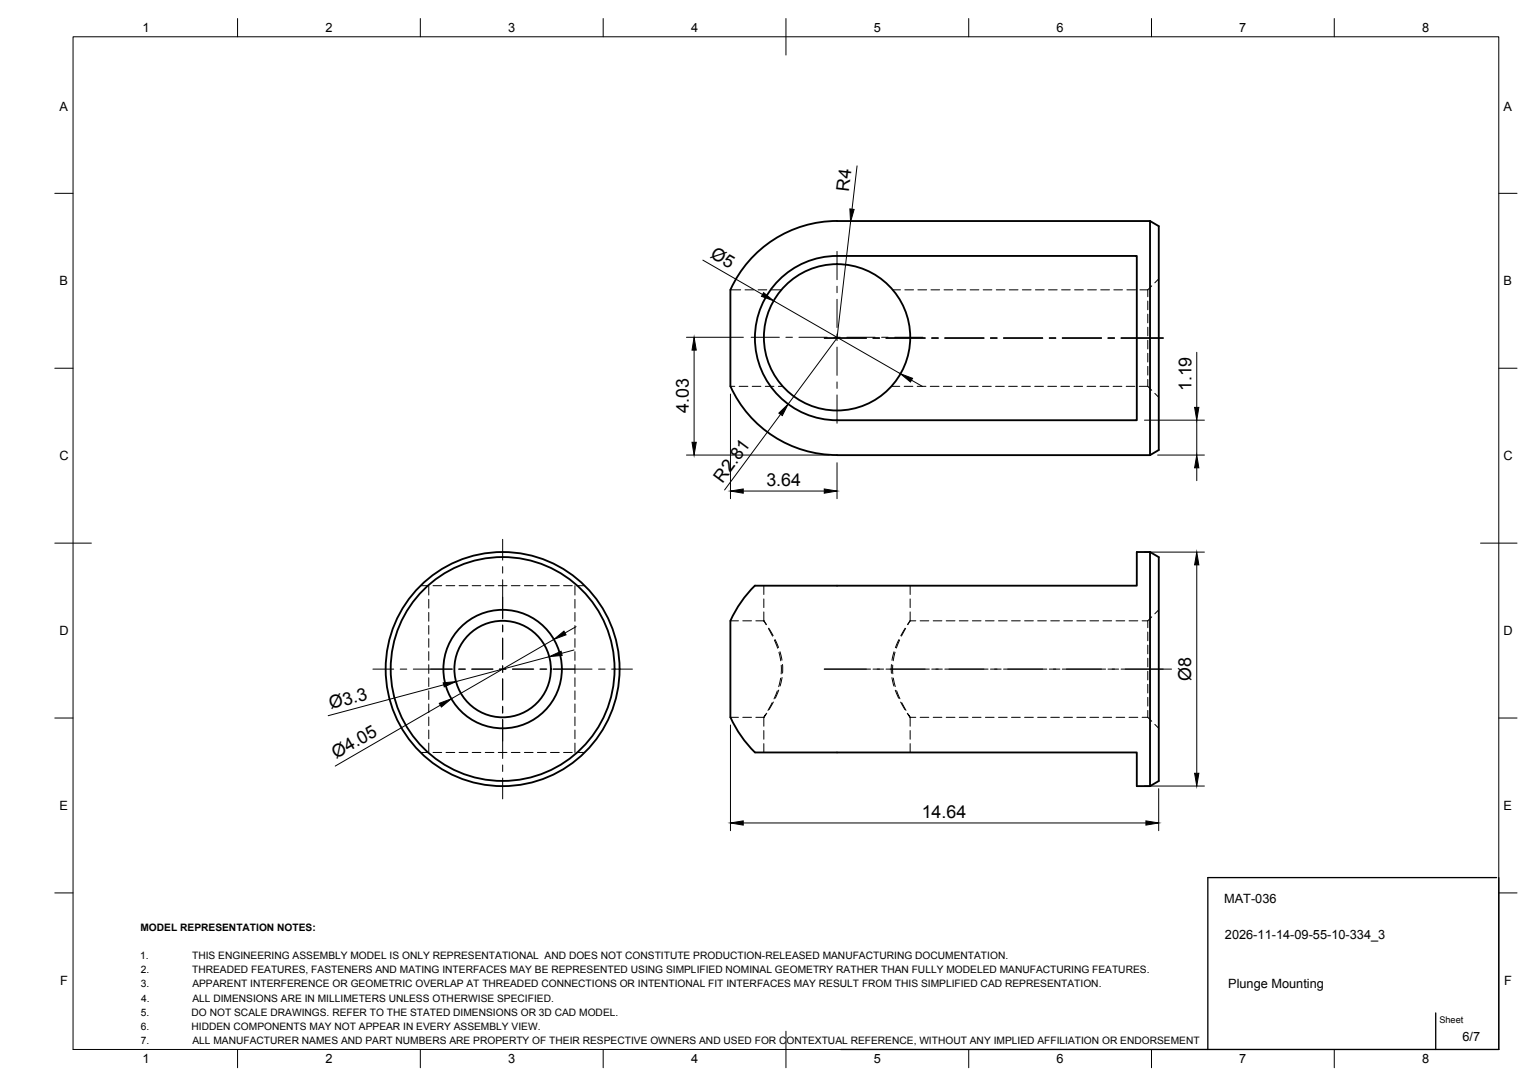
ISO-10303-21;
HEADER;
/* Generated by software containing ST-Developer
 * from STEP Tools, Inc. (www.steptools.com) 
 */

FILE_DESCRIPTION(
/* description */ (''),
/* implementation_level */ '2;1');

FILE_NAME(
/* name */ 'Plunge Mounting.step',
/* time_stamp */ '2026-11-14T09:55:16-08:00',
/* author */ (''),
/* organization */ (''),
/* preprocessor_version */ 'ST-DEVELOPER v20.2',
/* originating_system */ 'Autodesk Translation Framework v15.17.0.0',
/* authorisation */ '');

FILE_SCHEMA (('AUTOMOTIVE_DESIGN { 1 0 10303 214 3 1 1 }'));
ENDSEC;

DATA;
#10=MECHANICAL_DESIGN_GEOMETRIC_PRESENTATION_REPRESENTATION('',(#61),#170250);
#35=SPHERICAL_SURFACE('',#77715,4.00000000000002);
#47=SHAPE_REPRESENTATION_RELATIONSHIP('SRR','None',#170279,#53);
#53=ADVANCED_BREP_SHAPE_REPRESENTATION('',(#67),#170247);
#61=STYLED_ITEM('',(#170315),#67);
#67=MANIFOLD_SOLID_BREP('Body1',#71401);
#80=FACE_BOUND('',#15903,.T.);
#81=FACE_BOUND('',#15905,.T.);
#82=FACE_BOUND('',#15911,.T.);
#83=FACE_BOUND('',#15916,.T.);
#84=FACE_BOUND('',#15918,.T.);
#103=PLANE('',#77733);
#104=PLANE('',#77734);
#105=PLANE('',#77735);
#106=PLANE('',#77737);
#107=PLANE('',#77738);
#5376=CYLINDRICAL_SURFACE('',#77712,2.5);
#5377=CYLINDRICAL_SURFACE('',#77722,4.);
#5378=CYLINDRICAL_SURFACE('',#77732,1.65);
#5379=CYLINDRICAL_SURFACE('',#77736,1.65);
#10627=FACE_OUTER_BOUND('',#15902,.T.);
#10628=FACE_OUTER_BOUND('',#15904,.T.);
#10629=FACE_OUTER_BOUND('',#15906,.T.);
#10630=FACE_OUTER_BOUND('',#15907,.T.);
#10631=FACE_OUTER_BOUND('',#15908,.T.);
#10632=FACE_OUTER_BOUND('',#15909,.T.);
#10633=FACE_OUTER_BOUND('',#15910,.T.);
#10634=FACE_OUTER_BOUND('',#15912,.T.);
#10635=FACE_OUTER_BOUND('',#15913,.T.);
#10636=FACE_OUTER_BOUND('',#15914,.T.);
#10637=FACE_OUTER_BOUND('',#15915,.T.);
#10638=FACE_OUTER_BOUND('',#15917,.T.);
#15902=EDGE_LOOP('',(#65902,#65903,#65904,#65905,#65906,#65907,#65908,#65909,
#65910));
#15903=EDGE_LOOP('',(#65911,#65912));
#15904=EDGE_LOOP('',(#65913,#65914,#65915,#65916,#65917));
#15905=EDGE_LOOP('',(#65918));
#15906=EDGE_LOOP('',(#65919,#65920,#65921,#65922,#65923,#65924,#65925,#65926,
#65927,#65928,#65929,#65930,#65931));
#15907=EDGE_LOOP('',(#65932,#65933,#65934,#65935));
#15908=EDGE_LOOP('',(#65936,#65937,#65938,#65939,#65940));
#15909=EDGE_LOOP('',(#65941,#65942,#65943,#65944,#65945));
#15910=EDGE_LOOP('',(#65946));
#15911=EDGE_LOOP('',(#65947));
#15912=EDGE_LOOP('',(#65948,#65949));
#15913=EDGE_LOOP('',(#65950,#65951));
#15914=EDGE_LOOP('',(#65952,#65953,#65954,#65955,#65956,#65957));
#15915=EDGE_LOOP('',(#65958,#65959,#65960,#65961));
#15916=EDGE_LOOP('',(#65962));
#15917=EDGE_LOOP('',(#65963,#65964,#65965,#65966));
#15918=EDGE_LOOP('',(#65967));
#21024=CIRCLE('',#77713,2.5);
#21025=CIRCLE('',#77714,2.5);
#21026=CIRCLE('',#77716,3.9999999997442);
#21027=CIRCLE('',#77717,2.80668844013728);
#21028=CIRCLE('',#77718,3.9999999997442);
#21029=CIRCLE('',#77719,3.9999999997442);
#21030=CIRCLE('',#77720,2.80668844013726);
#21031=CIRCLE('',#77721,1.64999996202742);
#21032=CIRCLE('',#77723,4.);
#21033=CIRCLE('',#77724,4.);
#21034=CIRCLE('',#77725,4.);
#21035=CIRCLE('',#77726,4.);
#21036=CIRCLE('',#77728,1.65);
#21037=CIRCLE('',#77729,2.025);
#21038=CIRCLE('',#77731,3.826794919);
#24347=B_SPLINE_CURVE_WITH_KNOTS('',3,(#169973,#169974,#169975,#169976,
#169977,#169978,#169979,#169980,#169981,#169982,#169983,#169984,#169985,
#169986,#169987,#169988,#169989,#169990),.UNSPECIFIED.,.F.,.F.,(4,2,2,2,
2,2,2,2,4),(-0.772891272014126,-0.711371011943309,-0.647238677062543,-0.582315553959231,
-0.517392430855918,-0.452469307752605,-0.387546184649291,-0.323413849768526,
-0.261893589697701),.UNSPECIFIED.);
#24348=B_SPLINE_CURVE_WITH_KNOTS('',3,(#169995,#169996,#169997,#169998),
 .UNSPECIFIED.,.F.,.F.,(4,4),(-0.261893589697701,-0.25928151488776),
 .UNSPECIFIED.);
#24349=B_SPLINE_CURVE_WITH_KNOTS('',3,(#169999,#170000,#170001,#170002,
#170003,#170004,#170005,#170006,#170007,#170008,#170009,#170010,#170011,
#170012,#170013,#170014,#170015,#170016,#170017,#170018,#170019),
 .UNSPECIFIED.,.F.,.F.,(4,2,2,2,3,2,2,2,2,4),(-0.25928151488776,-0.194741358681164,
-0.130201202474569,-0.0651006012372844,0.,0.0651006012372838,0.130201202474568,
0.194741358681163,0.259281514887759,0.261893589697708),.UNSPECIFIED.);
#24350=B_SPLINE_CURVE_WITH_KNOTS('',3,(#170022,#170023,#170024,#170025,
#170026,#170027,#170028,#170029,#170030,#170031),.UNSPECIFIED.,.F.,.F.,
(4,2,2,2,4),(-0.772891272014128,-0.711371011943309,-0.647238677062543,-0.58231555395923,
-0.517392430855917),.UNSPECIFIED.);
#24351=B_SPLINE_CURVE_WITH_KNOTS('',3,(#170032,#170033,#170034,#170035,
#170036,#170037,#170038,#170039,#170040,#170041,#170042,#170043,#170044,
#170045,#170046,#170047,#170048,#170049,#170050,#170051,#170052,#170053,
#170054,#170055,#170056,#170057,#170058,#170059,#170060),.UNSPECIFIED.,
 .F.,.F.,(4,2,2,2,2,2,2,2,3,2,2,2,2,4),(-0.517392430855917,-0.452469307752604,
-0.38754618464929,-0.323413849768524,-0.259281514887758,-0.194741358681163,
-0.130201202474568,-0.0651006012372838,0.,0.0651694580098041,0.130338916019608,
0.194810907043524,0.25928289806744,0.261894972877388),.UNSPECIFIED.);
#26426=LINE('',#169971,#28514);
#26427=LINE('',#169992,#28515);
#26428=LINE('',#170079,#28516);
#26429=LINE('',#170081,#28517);
#26430=LINE('',#170084,#28518);
#26431=LINE('',#170086,#28519);
#26432=LINE('',#170089,#28520);
#26433=LINE('',#170094,#28521);
#26434=LINE('',#170098,#28522);
#26435=LINE('',#170101,#28523);
#26436=LINE('',#170104,#28524);
#26437=LINE('',#170106,#28525);
#26438=LINE('',#170108,#28526);
#28514=VECTOR('',#92318,2.5);
#28515=VECTOR('',#92319,2.5);
#28516=VECTOR('',#92342,4.);
#28517=VECTOR('',#92343,1000.);
#28518=VECTOR('',#92346,1000.);
#28519=VECTOR('',#92347,1000.);
#28520=VECTOR('',#92350,1000.);
#28521=VECTOR('',#92355,1.65);
#28522=VECTOR('',#92360,3.826794919);
#28523=VECTOR('',#92365,1.65);
#28524=VECTOR('',#92370,1000.);
#28525=VECTOR('',#92373,1000.);
#28526=VECTOR('',#92376,1.65);
#33930=VERTEX_POINT('',#169968);
#33931=VERTEX_POINT('',#169970);
#33932=VERTEX_POINT('',#169972);
#33933=VERTEX_POINT('',#169991);
#33934=VERTEX_POINT('',#169994);
#33935=VERTEX_POINT('',#170020);
#33936=VERTEX_POINT('',#170021);
#33937=VERTEX_POINT('',#170062);
#33938=VERTEX_POINT('',#170063);
#33939=VERTEX_POINT('',#170065);
#33940=VERTEX_POINT('',#170067);
#33941=VERTEX_POINT('',#170069);
#33942=VERTEX_POINT('',#170072);
#33943=VERTEX_POINT('',#170075);
#33944=VERTEX_POINT('',#170076);
#33945=VERTEX_POINT('',#170080);
#33946=VERTEX_POINT('',#170082);
#33947=VERTEX_POINT('',#170085);
#33948=VERTEX_POINT('',#170087);
#33949=VERTEX_POINT('',#170091);
#33950=VERTEX_POINT('',#170093);
#33951=VERTEX_POINT('',#170097);
#44595=EDGE_CURVE('',#33930,#33930,#21024,.T.);
#44596=EDGE_CURVE('',#33930,#33931,#26426,.T.);
#44597=EDGE_CURVE('',#33931,#33932,#24347,.T.);
#44598=EDGE_CURVE('',#33932,#33933,#26427,.T.);
#44599=EDGE_CURVE('',#33933,#33933,#21025,.T.);
#44600=EDGE_CURVE('',#33932,#33934,#24348,.T.);
#44601=EDGE_CURVE('',#33934,#33931,#24349,.T.);
#44602=EDGE_CURVE('',#33935,#33936,#24350,.T.);
#44603=EDGE_CURVE('',#33936,#33935,#24351,.T.);
#44604=EDGE_CURVE('',#33937,#33938,#21026,.T.);
#44605=EDGE_CURVE('',#33937,#33939,#21027,.T.);
#44606=EDGE_CURVE('',#33940,#33939,#21028,.T.);
#44607=EDGE_CURVE('',#33941,#33940,#21029,.T.);
#44608=EDGE_CURVE('',#33941,#33938,#21030,.T.);
#44609=EDGE_CURVE('',#33942,#33942,#21031,.T.);
#44610=EDGE_CURVE('',#33943,#33944,#21032,.T.);
#44611=EDGE_CURVE('',#33944,#33943,#21033,.T.);
#44612=EDGE_CURVE('',#33944,#33940,#26428,.T.);
#44613=EDGE_CURVE('',#33939,#33945,#26429,.T.);
#44614=EDGE_CURVE('',#33946,#33945,#21034,.T.);
#44615=EDGE_CURVE('',#33946,#33937,#26430,.T.);
#44616=EDGE_CURVE('',#33938,#33947,#26431,.T.);
#44617=EDGE_CURVE('',#33948,#33947,#21035,.T.);
#44618=EDGE_CURVE('',#33948,#33941,#26432,.T.);
#44619=EDGE_CURVE('',#33949,#33949,#21036,.T.);
#44620=EDGE_CURVE('',#33949,#33950,#26433,.T.);
#44621=EDGE_CURVE('',#33950,#33950,#21037,.T.);
#44622=EDGE_CURVE('',#33943,#33951,#26434,.T.);
#44623=EDGE_CURVE('',#33951,#33951,#21038,.T.);
#44624=EDGE_CURVE('',#33936,#33949,#26435,.T.);
#44625=EDGE_CURVE('',#33945,#33946,#26436,.T.);
#44626=EDGE_CURVE('',#33947,#33948,#26437,.T.);
#44627=EDGE_CURVE('',#33942,#33934,#26438,.T.);
#65902=ORIENTED_EDGE('',*,*,#44595,.T.);
#65903=ORIENTED_EDGE('',*,*,#44596,.T.);
#65904=ORIENTED_EDGE('',*,*,#44597,.T.);
#65905=ORIENTED_EDGE('',*,*,#44598,.T.);
#65906=ORIENTED_EDGE('',*,*,#44599,.T.);
#65907=ORIENTED_EDGE('',*,*,#44598,.F.);
#65908=ORIENTED_EDGE('',*,*,#44600,.T.);
#65909=ORIENTED_EDGE('',*,*,#44601,.T.);
#65910=ORIENTED_EDGE('',*,*,#44596,.F.);
#65911=ORIENTED_EDGE('',*,*,#44602,.T.);
#65912=ORIENTED_EDGE('',*,*,#44603,.T.);
#65913=ORIENTED_EDGE('',*,*,#44604,.F.);
#65914=ORIENTED_EDGE('',*,*,#44605,.T.);
#65915=ORIENTED_EDGE('',*,*,#44606,.F.);
#65916=ORIENTED_EDGE('',*,*,#44607,.F.);
#65917=ORIENTED_EDGE('',*,*,#44608,.T.);
#65918=ORIENTED_EDGE('',*,*,#44609,.F.);
#65919=ORIENTED_EDGE('',*,*,#44610,.F.);
#65920=ORIENTED_EDGE('',*,*,#44611,.F.);
#65921=ORIENTED_EDGE('',*,*,#44612,.T.);
#65922=ORIENTED_EDGE('',*,*,#44606,.T.);
#65923=ORIENTED_EDGE('',*,*,#44613,.T.);
#65924=ORIENTED_EDGE('',*,*,#44614,.F.);
#65925=ORIENTED_EDGE('',*,*,#44615,.T.);
#65926=ORIENTED_EDGE('',*,*,#44604,.T.);
#65927=ORIENTED_EDGE('',*,*,#44616,.T.);
#65928=ORIENTED_EDGE('',*,*,#44617,.F.);
#65929=ORIENTED_EDGE('',*,*,#44618,.T.);
#65930=ORIENTED_EDGE('',*,*,#44607,.T.);
#65931=ORIENTED_EDGE('',*,*,#44612,.F.);
#65932=ORIENTED_EDGE('',*,*,#44619,.F.);
#65933=ORIENTED_EDGE('',*,*,#44620,.T.);
#65934=ORIENTED_EDGE('',*,*,#44621,.T.);
#65935=ORIENTED_EDGE('',*,*,#44620,.F.);
#65936=ORIENTED_EDGE('',*,*,#44610,.T.);
#65937=ORIENTED_EDGE('',*,*,#44611,.T.);
#65938=ORIENTED_EDGE('',*,*,#44622,.T.);
#65939=ORIENTED_EDGE('',*,*,#44623,.F.);
#65940=ORIENTED_EDGE('',*,*,#44622,.F.);
#65941=ORIENTED_EDGE('',*,*,#44602,.F.);
#65942=ORIENTED_EDGE('',*,*,#44603,.F.);
#65943=ORIENTED_EDGE('',*,*,#44624,.T.);
#65944=ORIENTED_EDGE('',*,*,#44619,.T.);
#65945=ORIENTED_EDGE('',*,*,#44624,.F.);
#65946=ORIENTED_EDGE('',*,*,#44623,.T.);
#65947=ORIENTED_EDGE('',*,*,#44621,.F.);
#65948=ORIENTED_EDGE('',*,*,#44625,.T.);
#65949=ORIENTED_EDGE('',*,*,#44614,.T.);
#65950=ORIENTED_EDGE('',*,*,#44626,.T.);
#65951=ORIENTED_EDGE('',*,*,#44617,.T.);
#65952=ORIENTED_EDGE('',*,*,#44609,.T.);
#65953=ORIENTED_EDGE('',*,*,#44627,.T.);
#65954=ORIENTED_EDGE('',*,*,#44600,.F.);
#65955=ORIENTED_EDGE('',*,*,#44597,.F.);
#65956=ORIENTED_EDGE('',*,*,#44601,.F.);
#65957=ORIENTED_EDGE('',*,*,#44627,.F.);
#65958=ORIENTED_EDGE('',*,*,#44615,.F.);
#65959=ORIENTED_EDGE('',*,*,#44625,.F.);
#65960=ORIENTED_EDGE('',*,*,#44613,.F.);
#65961=ORIENTED_EDGE('',*,*,#44605,.F.);
#65962=ORIENTED_EDGE('',*,*,#44595,.F.);
#65963=ORIENTED_EDGE('',*,*,#44618,.F.);
#65964=ORIENTED_EDGE('',*,*,#44626,.F.);
#65965=ORIENTED_EDGE('',*,*,#44616,.F.);
#65966=ORIENTED_EDGE('',*,*,#44608,.F.);
#65967=ORIENTED_EDGE('',*,*,#44599,.F.);
#66129=CONICAL_SURFACE('',#77727,1.65,0.785398163397448);
#66130=CONICAL_SURFACE('',#77730,3.826794919,0.52359877620608);
#71377=ADVANCED_FACE('',(#10627,#80),#5376,.F.);
#71378=ADVANCED_FACE('',(#10628,#81),#35,.T.);
#71379=ADVANCED_FACE('',(#10629),#5377,.T.);
#71380=ADVANCED_FACE('',(#10630),#66129,.F.);
#71381=ADVANCED_FACE('',(#10631),#66130,.T.);
#71382=ADVANCED_FACE('',(#10632),#5378,.F.);
#71383=ADVANCED_FACE('',(#10633,#82),#103,.T.);
#71384=ADVANCED_FACE('',(#10634),#104,.F.);
#71385=ADVANCED_FACE('',(#10635),#105,.F.);
#71386=ADVANCED_FACE('',(#10636),#5379,.F.);
#71387=ADVANCED_FACE('',(#10637,#83),#106,.F.);
#71388=ADVANCED_FACE('',(#10638,#84),#107,.F.);
#71401=CLOSED_SHELL('',(#71377,#71378,#71379,#71380,#71381,#71382,#71383,
#71384,#71385,#71386,#71387,#71388));
#77711=AXIS2_PLACEMENT_3D('',#169966,#92312,#92313);
#77712=AXIS2_PLACEMENT_3D('',#169967,#92314,#92315);
#77713=AXIS2_PLACEMENT_3D('',#169969,#92316,#92317);
#77714=AXIS2_PLACEMENT_3D('',#169993,#92320,#92321);
#77715=AXIS2_PLACEMENT_3D('',#170061,#92322,#92323);
#77716=AXIS2_PLACEMENT_3D('',#170064,#92324,#92325);
#77717=AXIS2_PLACEMENT_3D('',#170066,#92326,#92327);
#77718=AXIS2_PLACEMENT_3D('',#170068,#92328,#92329);
#77719=AXIS2_PLACEMENT_3D('',#170070,#92330,#92331);
#77720=AXIS2_PLACEMENT_3D('',#170071,#92332,#92333);
#77721=AXIS2_PLACEMENT_3D('',#170073,#92334,#92335);
#77722=AXIS2_PLACEMENT_3D('',#170074,#92336,#92337);
#77723=AXIS2_PLACEMENT_3D('',#170077,#92338,#92339);
#77724=AXIS2_PLACEMENT_3D('',#170078,#92340,#92341);
#77725=AXIS2_PLACEMENT_3D('',#170083,#92344,#92345);
#77726=AXIS2_PLACEMENT_3D('',#170088,#92348,#92349);
#77727=AXIS2_PLACEMENT_3D('',#170090,#92351,#92352);
#77728=AXIS2_PLACEMENT_3D('',#170092,#92353,#92354);
#77729=AXIS2_PLACEMENT_3D('',#170095,#92356,#92357);
#77730=AXIS2_PLACEMENT_3D('',#170096,#92358,#92359);
#77731=AXIS2_PLACEMENT_3D('',#170099,#92361,#92362);
#77732=AXIS2_PLACEMENT_3D('',#170100,#92363,#92364);
#77733=AXIS2_PLACEMENT_3D('',#170102,#92366,#92367);
#77734=AXIS2_PLACEMENT_3D('',#170103,#92368,#92369);
#77735=AXIS2_PLACEMENT_3D('',#170105,#92371,#92372);
#77736=AXIS2_PLACEMENT_3D('',#170107,#92374,#92375);
#77737=AXIS2_PLACEMENT_3D('',#170109,#92377,#92378);
#77738=AXIS2_PLACEMENT_3D('',#170110,#92379,#92380);
#92312=DIRECTION('axis',(0.,0.,1.));
#92313=DIRECTION('refdir',(1.,0.,0.));
#92314=DIRECTION('center_axis',(0.,3.46944695195361E-16,1.));
#92315=DIRECTION('ref_axis',(0.,-1.,3.46944695195361E-16));
#92316=DIRECTION('center_axis',(0.,-3.46944695195361E-16,-1.));
#92317=DIRECTION('ref_axis',(0.,-1.,3.46944695195361E-16));
#92318=DIRECTION('',(0.,3.46944695195361E-16,1.));
#92319=DIRECTION('',(0.,3.46944695195361E-16,1.));
#92320=DIRECTION('center_axis',(0.,3.46944695195361E-16,1.));
#92321=DIRECTION('ref_axis',(0.,-1.,3.46944695195361E-16));
#92322=DIRECTION('center_axis',(1.20172968798293E-14,-7.54951656745103E-15,
1.));
#92323=DIRECTION('ref_axis',(1.,0.,-1.19556786944265E-14));
#92324=DIRECTION('center_axis',(0.,-1.,0.));
#92325=DIRECTION('ref_axis',(1.,0.,-6.98296267747417E-15));
#92326=DIRECTION('center_axis',(0.,0.,1.));
#92327=DIRECTION('ref_axis',(1.,0.,0.));
#92328=DIRECTION('center_axis',(0.,-1.,0.));
#92329=DIRECTION('ref_axis',(1.,0.,-6.98296267747417E-15));
#92330=DIRECTION('center_axis',(0.,-1.,0.));
#92331=DIRECTION('ref_axis',(1.,0.,-6.98296267747417E-15));
#92332=DIRECTION('center_axis',(0.,0.,-1.));
#92333=DIRECTION('ref_axis',(-1.,0.,0.));
#92334=DIRECTION('center_axis',(0.,1.,0.));
#92335=DIRECTION('ref_axis',(1.,0.,-6.98296267717208E-15));
#92336=DIRECTION('center_axis',(-2.22101865678853E-15,-1.,2.2210186565311E-15));
#92337=DIRECTION('ref_axis',(1.,-2.22101865678853E-15,1.16857368147256E-31));
#92338=DIRECTION('center_axis',(0.,-1.,-1.23599047663347E-14));
#92339=DIRECTION('ref_axis',(0.,-1.23599047663347E-14,1.));
#92340=DIRECTION('center_axis',(0.,-1.,-1.23599047663347E-14));
#92341=DIRECTION('ref_axis',(0.,-1.23599047663347E-14,1.));
#92342=DIRECTION('',(2.22101865678853E-15,1.,-2.2210186565311E-15));
#92343=DIRECTION('',(0.,-1.,0.));
#92344=DIRECTION('center_axis',(2.22101865678853E-15,1.,-2.2210186565311E-15));
#92345=DIRECTION('ref_axis',(1.,-2.22101865678853E-15,1.16857368147256E-31));
#92346=DIRECTION('',(0.,1.,0.));
#92347=DIRECTION('',(0.,-1.,0.));
#92348=DIRECTION('center_axis',(2.22101865678853E-15,1.,-2.2210186565311E-15));
#92349=DIRECTION('ref_axis',(1.,-2.22101865678853E-15,1.16857368147256E-31));
#92350=DIRECTION('',(0.,1.,0.));
#92351=DIRECTION('center_axis',(-1.31418445149758E-16,-1.,0.));
#92352=DIRECTION('ref_axis',(1.,-1.31418445149758E-16,0.));
#92353=DIRECTION('center_axis',(0.,-1.,0.));
#92354=DIRECTION('ref_axis',(0.,0.,-1.));
#92355=DIRECTION('',(-0.707106781186547,-0.707106781186547,-8.65956056235493E-17));
#92356=DIRECTION('center_axis',(0.,-1.,0.));
#92357=DIRECTION('ref_axis',(0.,0.,-1.));
#92358=DIRECTION('center_axis',(-1.13327439325526E-16,1.,0.));
#92359=DIRECTION('ref_axis',(-1.,-1.13327439325526E-16,0.));
#92360=DIRECTION('',(-0.500000000526354,-0.866025403480548,6.12323400218274E-17));
#92361=DIRECTION('center_axis',(0.,-1.,0.));
#92362=DIRECTION('ref_axis',(0.,0.,1.));
#92363=DIRECTION('center_axis',(7.17905020235292E-15,-1.,-7.17905020184743E-15));
#92364=DIRECTION('ref_axis',(1.,7.17905020235292E-15,-1.29497664574085E-30));
#92365=DIRECTION('',(7.17905020235292E-15,-1.,-7.17905020184743E-15));
#92366=DIRECTION('center_axis',(0.,-1.,0.));
#92367=DIRECTION('ref_axis',(0.,0.,-1.));
#92368=DIRECTION('center_axis',(0.,-1.,0.));
#92369=DIRECTION('ref_axis',(0.,0.,-1.));
#92370=DIRECTION('',(1.,0.,0.));
#92371=DIRECTION('center_axis',(0.,-1.,0.));
#92372=DIRECTION('ref_axis',(0.,0.,-1.));
#92373=DIRECTION('',(-1.,0.,0.));
#92374=DIRECTION('center_axis',(1.4358100401433E-14,-1.,-1.43581004053009E-14));
#92375=DIRECTION('ref_axis',(5.17990657360398E-30,1.43581004053009E-14,
-1.));
#92376=DIRECTION('',(1.4358100401433E-14,-1.,-1.43581004053009E-14));
#92377=DIRECTION('center_axis',(0.,0.,1.));
#92378=DIRECTION('ref_axis',(1.,0.,0.));
#92379=DIRECTION('center_axis',(0.,0.,-1.));
#92380=DIRECTION('ref_axis',(0.,-1.,0.));
#169966=CARTESIAN_POINT('',(0.,0.,0.));
#169967=CARTESIAN_POINT('Origin',(0.,13.199314767,-2.85));
#169968=CARTESIAN_POINT('',(-3.06161699786838E-16,15.699314767,-2.85));
#169969=CARTESIAN_POINT('Origin',(0.,13.199314767,-2.85));
#169970=CARTESIAN_POINT('',(-8.13037459096346E-14,15.699314767,-1.64979248298911));
#169971=CARTESIAN_POINT('',(-3.06161699786838E-16,15.699314767,-2.85));
#169972=CARTESIAN_POINT('',(-1.48881792639556E-15,15.699314767,1.6497924829891));
#169973=CARTESIAN_POINT('Ctrl Pts',(-8.00401411815699E-14,15.699314767,
-1.64979248298913));
#169974=CARTESIAN_POINT('Ctrl Pts',(-0.205803259960164,15.699314767,-1.64652816021247));
#169975=CARTESIAN_POINT('Ctrl Pts',(-0.419768902376369,15.6719454978376,
-1.60250021812967));
#169976=CARTESIAN_POINT('Ctrl Pts',(-0.816290167466643,15.5714988188155,
-1.43561074613428));
#169977=CARTESIAN_POINT('Ctrl Pts',(-0.997484282319592,15.4972611642841,
-1.30959123284094));
#169978=CARTESIAN_POINT('Ctrl Pts',(-1.28367540143835,15.3506733018643,
-1.02381919842138));
#169979=CARTESIAN_POINT('Ctrl Pts',(-1.40913392628232,15.2670643837886,
-0.842787202998243));
#169980=CARTESIAN_POINT('Ctrl Pts',(-1.57919184577488,15.1402942605532,
-0.439545146879724));
#169981=CARTESIAN_POINT('Ctrl Pts',(-1.62383202199997,15.1001486798728,
-0.216410410344402));
#169982=CARTESIAN_POINT('Ctrl Pts',(-1.62383202199997,15.1001486798728,
0.216410410344351));
#169983=CARTESIAN_POINT('Ctrl Pts',(-1.57919184577488,15.1402942605532,
0.439545146879674));
#169984=CARTESIAN_POINT('Ctrl Pts',(-1.40913392628232,15.2670643837886,
0.842787202998197));
#169985=CARTESIAN_POINT('Ctrl Pts',(-1.28367540143835,15.3506733018643,
1.02381919842134));
#169986=CARTESIAN_POINT('Ctrl Pts',(-0.99748428231959,15.4972611642841,
1.3095912328409));
#169987=CARTESIAN_POINT('Ctrl Pts',(-0.816290167466642,15.5714988188155,
1.43561074613424));
#169988=CARTESIAN_POINT('Ctrl Pts',(-0.419768902376345,15.6719454978376,
1.60250021812965));
#169989=CARTESIAN_POINT('Ctrl Pts',(-0.20580325996011,15.699314767,1.64652816021244));
#169990=CARTESIAN_POINT('Ctrl Pts',(-2.46330733588707E-15,15.699314767,
1.6497924829891));
#169991=CARTESIAN_POINT('',(-3.06161699786838E-16,15.699314767,2.85));
#169992=CARTESIAN_POINT('',(-3.06161699786838E-16,15.699314767,-2.85));
#169993=CARTESIAN_POINT('Origin',(0.,13.199314767,2.85));
#169994=CARTESIAN_POINT('',(0.0261679780000193,15.6991778106341,1.64999999999998));
#169995=CARTESIAN_POINT('Ctrl Pts',(-2.60556586232155E-15,15.699314767,
1.6497924829891));
#169996=CARTESIAN_POINT('Ctrl Pts',(0.00873815407357623,15.699314767,1.64993108213166));
#169997=CARTESIAN_POINT('Ctrl Pts',(0.0174615389539147,15.699268947589,
1.64999999999998));
#169998=CARTESIAN_POINT('Ctrl Pts',(0.0261679780000195,15.6991778106341,
1.64999999999998));
#169999=CARTESIAN_POINT('Ctrl Pts',(0.0261679780000195,15.6991778106341,
1.64999999999998));
#170000=CARTESIAN_POINT('Ctrl Pts',(0.241290046441671,15.6969259634504,
1.64999999999998));
#170001=CARTESIAN_POINT('Ctrl Pts',(0.465876783427725,15.664501349548,1.60546249013418));
#170002=CARTESIAN_POINT('Ctrl Pts',(0.870980543861273,15.5520958562483,
1.43427513780378));
#170003=CARTESIAN_POINT('Ctrl Pts',(1.05188113671723,15.4729968985576,1.30795540755756));
#170004=CARTESIAN_POINT('Ctrl Pts',(1.33692048386355,15.3180839765991,1.02248044003066));
#170005=CARTESIAN_POINT('Ctrl Pts',(1.46178671653895,15.2302813588062,0.842103770333563));
#170006=CARTESIAN_POINT('Ctrl Pts',(1.63136593636146,15.0967583709211,0.439861055965033));
#170007=CARTESIAN_POINT('Ctrl Pts',(1.67616797800003,15.0541627148187,0.217002004124254));
#170008=CARTESIAN_POINT('Ctrl Pts',(1.67616797800003,15.0541627148187,-2.72004641033163E-14));
#170009=CARTESIAN_POINT('Ctrl Pts',(1.67616797800003,15.0541627148187,-0.217002004124306));
#170010=CARTESIAN_POINT('Ctrl Pts',(1.63136593636147,15.0967583709211,-0.439861055965085));
#170011=CARTESIAN_POINT('Ctrl Pts',(1.46178671653895,15.2302813588062,-0.84210377033361));
#170012=CARTESIAN_POINT('Ctrl Pts',(1.33692048386356,15.3180839765991,-1.02248044003071));
#170013=CARTESIAN_POINT('Ctrl Pts',(1.05188113671723,15.4729968985576,-1.3079554075576));
#170014=CARTESIAN_POINT('Ctrl Pts',(0.870980543861275,15.5520958562483,
-1.43427513780382));
#170015=CARTESIAN_POINT('Ctrl Pts',(0.465876783427725,15.664501349548,-1.60546249013422));
#170016=CARTESIAN_POINT('Ctrl Pts',(0.241290046441671,15.6969259634504,
-1.65000000000002));
#170017=CARTESIAN_POINT('Ctrl Pts',(0.0174615389538886,15.699268947589,
-1.65000000000002));
#170018=CARTESIAN_POINT('Ctrl Pts',(0.00873815407352446,15.699314767,-1.6499310821317));
#170019=CARTESIAN_POINT('Ctrl Pts',(-8.00931456293832E-14,15.699314767,
-1.64979248298913));
#170020=CARTESIAN_POINT('',(-8.13936089372119E-14,10.699314767,1.64979248298911));
#170021=CARTESIAN_POINT('',(-1.623832022,11.2984808541272,-1.63563501057272E-15));
#170022=CARTESIAN_POINT('Ctrl Pts',(-7.96238075473354E-14,10.699314767,
1.64979248298911));
#170023=CARTESIAN_POINT('Ctrl Pts',(-0.205803259960169,10.699314767,1.64652816021245));
#170024=CARTESIAN_POINT('Ctrl Pts',(-0.41976890237638,10.7266840361624,
1.60250021812965));
#170025=CARTESIAN_POINT('Ctrl Pts',(-0.81629016746666,10.8271307151845,
1.43561074613426));
#170026=CARTESIAN_POINT('Ctrl Pts',(-0.99748428231961,10.9013683697159,
1.30959123284092));
#170027=CARTESIAN_POINT('Ctrl Pts',(-1.28367540143837,11.0479562321357,
1.02381919842136));
#170028=CARTESIAN_POINT('Ctrl Pts',(-1.40913392628234,11.1315651502115,
0.842787202998217));
#170029=CARTESIAN_POINT('Ctrl Pts',(-1.57919184577491,11.2583352734469,
0.439545146879698));
#170030=CARTESIAN_POINT('Ctrl Pts',(-1.623832022,11.2984808541272,0.216410410344375));
#170031=CARTESIAN_POINT('Ctrl Pts',(-1.623832022,11.2984808541272,-1.38777878078145E-15));
#170032=CARTESIAN_POINT('Ctrl Pts',(-1.623832022,11.2984808541272,-1.76941794549634E-15));
#170033=CARTESIAN_POINT('Ctrl Pts',(-1.623832022,11.2984808541272,-0.216410410344379));
#170034=CARTESIAN_POINT('Ctrl Pts',(-1.57919184577491,11.2583352734469,
-0.439545146879702));
#170035=CARTESIAN_POINT('Ctrl Pts',(-1.40913392628234,11.1315651502115,
-0.842787202998223));
#170036=CARTESIAN_POINT('Ctrl Pts',(-1.28367540143837,11.0479562321357,
-1.02381919842136));
#170037=CARTESIAN_POINT('Ctrl Pts',(-0.997484282319612,10.9013683697159,
-1.30959123284092));
#170038=CARTESIAN_POINT('Ctrl Pts',(-0.816290167466661,10.8271307151845,
-1.43561074613427));
#170039=CARTESIAN_POINT('Ctrl Pts',(-0.411525990970135,10.7245959436712,
-1.60596952798365));
#170040=CARTESIAN_POINT('Ctrl Pts',(-0.187594760493849,10.6972141053283,
-1.65));
#170041=CARTESIAN_POINT('Ctrl Pts',(0.241290046441657,10.7017035705496,
-1.65));
#170042=CARTESIAN_POINT('Ctrl Pts',(0.46587678342771,10.734128184452,-1.60546249013421));
#170043=CARTESIAN_POINT('Ctrl Pts',(0.870980543861256,10.8465336777517,
-1.4342751378038));
#170044=CARTESIAN_POINT('Ctrl Pts',(1.05188113671721,10.9256326354424,-1.30795540755759));
#170045=CARTESIAN_POINT('Ctrl Pts',(1.33692048386353,11.0805455574009,-1.02248044003069));
#170046=CARTESIAN_POINT('Ctrl Pts',(1.46178671653893,11.1683481751938,-0.84210377033359));
#170047=CARTESIAN_POINT('Ctrl Pts',(1.63136593636144,11.3018711630789,-0.439861055965061));
#170048=CARTESIAN_POINT('Ctrl Pts',(1.676167978,11.3444668191813,-0.217002004124281));
#170049=CARTESIAN_POINT('Ctrl Pts',(1.676167978,11.3444668191813,-1.66533453693773E-15));
#170050=CARTESIAN_POINT('Ctrl Pts',(1.676167978,11.3444668191813,0.217231526699345));
#170051=CARTESIAN_POINT('Ctrl Pts',(1.63127512468089,11.301782403439,0.440292498024009));
#170052=CARTESIAN_POINT('Ctrl Pts',(1.46138411208521,11.1680484789012,0.842842081218013));
#170053=CARTESIAN_POINT('Ctrl Pts',(1.33629461722267,11.0801303618484,1.02332573869294));
#170054=CARTESIAN_POINT('Ctrl Pts',(1.05102843990342,10.9252439245417,1.30859191601219));
#170055=CARTESIAN_POINT('Ctrl Pts',(0.870229942927133,10.84627169536,1.43468547107567));
#170056=CARTESIAN_POINT('Ctrl Pts',(0.465438353303639,10.7340604004941,
1.60555433928764));
#170057=CARTESIAN_POINT('Ctrl Pts',(0.241062841613601,10.7017011922229,
1.64999999999999));
#170058=CARTESIAN_POINT('Ctrl Pts',(0.0174615389538807,10.6993605864111,
1.64999999999999));
#170059=CARTESIAN_POINT('Ctrl Pts',(0.00873815407352076,10.699314767,1.64993108213168));
#170060=CARTESIAN_POINT('Ctrl Pts',(-7.97074750374294E-14,10.699314767,
1.64979248298911));
#170061=CARTESIAN_POINT('Origin',(0.0261679777441796,13.1993147672558,3.90673656623786E-24));
#170062=CARTESIAN_POINT('',(2.83285641798294,13.1993148047155,-2.84999999995817));
#170063=CARTESIAN_POINT('',(2.83285641847171,13.1993148047155,2.84999999986065));
#170064=CARTESIAN_POINT('Origin',(0.026167978,13.1993148064353,0.));
#170065=CARTESIAN_POINT('',(-2.7805204619831,13.1993148047155,-2.84999999995806));
#170066=CARTESIAN_POINT('Origin',(0.0261679782558256,13.1993147672558,-2.85));
#170067=CARTESIAN_POINT('',(-3.97383202200001,13.1993148064354,-1.00349951151754E-15));
#170068=CARTESIAN_POINT('Origin',(0.026167978,13.1993148064353,0.));
#170069=CARTESIAN_POINT('',(-2.78052046247155,13.1993148047155,2.84999999986076));
#170070=CARTESIAN_POINT('Origin',(0.026167978,13.1993148064353,0.));
#170071=CARTESIAN_POINT('Origin',(0.0261679777441796,13.1993147672558,2.85));
#170072=CARTESIAN_POINT('',(0.0261679774923747,16.8431451865352,1.64999996202742));
#170073=CARTESIAN_POINT('Origin',(0.026167978,16.8431451865352,0.));
#170074=CARTESIAN_POINT('Origin',(0.0261679779999925,13.199314767,-5.1364070427196E-16));
#170075=CARTESIAN_POINT('',(4.02616797800003,2.49931476700005,4.89858719658945E-16));
#170076=CARTESIAN_POINT('',(-3.97383202200003,2.499314767,2.2761400200952E-14));
#170077=CARTESIAN_POINT('Origin',(0.026167978,2.49931476700005,0.));
#170078=CARTESIAN_POINT('Origin',(0.026167978,2.49931476700005,0.));
#170079=CARTESIAN_POINT('',(-3.97383202200001,13.199314767,-1.0034994239309E-15));
#170080=CARTESIAN_POINT('',(-2.78052046215232,2.949314767,-2.85));
#170081=CARTESIAN_POINT('',(-2.78052046216742,2.949314767,-2.85));
#170082=CARTESIAN_POINT('',(2.8328564178964,2.949314767,-2.85));
#170083=CARTESIAN_POINT('Origin',(0.0261679779999697,2.94931476700001,2.22518005251719E-14));
#170084=CARTESIAN_POINT('',(2.8328564176556,2.949314767,-2.85));
#170085=CARTESIAN_POINT('',(2.83285641873687,2.949314767,2.85));
#170086=CARTESIAN_POINT('',(2.83285641933651,2.949314767,2.85));
#170087=CARTESIAN_POINT('',(-2.78052046248096,2.949314767,2.85));
#170088=CARTESIAN_POINT('Origin',(0.0261679779999697,2.949314767,2.22518005251719E-14));
#170089=CARTESIAN_POINT('',(-2.78052046282469,2.949314767,2.85));
#170090=CARTESIAN_POINT('Origin',(0.0261679779999999,2.574314767,0.));
#170091=CARTESIAN_POINT('',(-1.623832022,2.574314767,-2.02066721859313E-16));
#170092=CARTESIAN_POINT('Origin',(0.026167978,2.574314767,0.));
#170093=CARTESIAN_POINT('',(-1.99883202199996,2.19931476700004,-2.47990976827334E-16));
#170094=CARTESIAN_POINT('',(-1.623832022,2.574314767,-2.02066721859313E-16));
#170095=CARTESIAN_POINT('Origin',(0.026167978,2.19931476700008,0.));
#170096=CARTESIAN_POINT('Origin',(0.0261679780000002,2.199314767,0.));
#170097=CARTESIAN_POINT('',(3.85296289699999,2.19931476699998,-4.68647214854669E-16));
#170098=CARTESIAN_POINT('',(3.852962897,2.199314767,-4.68647214854671E-16));
#170099=CARTESIAN_POINT('Origin',(0.026167978,2.19931476699997,0.));
#170100=CARTESIAN_POINT('Origin',(0.0261679780000019,11.400319595,-9.15624615766385E-16));
#170101=CARTESIAN_POINT('',(-1.623832022,11.400319595,-1.1176913376257E-15));
#170102=CARTESIAN_POINT('Origin',(-3.84654848,2.199314767,3.872716458));
#170103=CARTESIAN_POINT('Origin',(-2.814200723,2.949314767,-2.85));
#170104=CARTESIAN_POINT('',(-2.814200723,2.949314767,-2.85));
#170105=CARTESIAN_POINT('Origin',(-2.814200723,2.949314767,4.0069));
#170106=CARTESIAN_POINT('',(-2.814200723,2.949314767,2.85));
#170107=CARTESIAN_POINT('Origin',(0.0261679780000029,16.84314517,-1.58198686873571E-15));
#170108=CARTESIAN_POINT('',(0.0261679780000027,16.8431451699999,1.65));
#170109=CARTESIAN_POINT('Origin',(-2.780520462,2.949314767,-2.85));
#170110=CARTESIAN_POINT('Origin',(2.832856418,2.949314767,2.85));
#170239=UNCERTAINTY_MEASURE_WITH_UNIT(LENGTH_MEASURE(0.01),#170251,
'DISTANCE_ACCURACY_VALUE',
'Maximum model space distance between geometric entities at asserted c
onnectivities');
#170242=UNCERTAINTY_MEASURE_WITH_UNIT(LENGTH_MEASURE(0.01),#170251,
'DISTANCE_ACCURACY_VALUE',
'Maximum model space distance between geometric entities at asserted c
onnectivities');
#170247=(
GEOMETRIC_REPRESENTATION_CONTEXT(3)
GLOBAL_UNCERTAINTY_ASSIGNED_CONTEXT((#170239))
GLOBAL_UNIT_ASSIGNED_CONTEXT((#170251,#170253,#170254))
REPRESENTATION_CONTEXT('','3D')
);
#170250=(
GEOMETRIC_REPRESENTATION_CONTEXT(3)
GLOBAL_UNCERTAINTY_ASSIGNED_CONTEXT((#170242))
GLOBAL_UNIT_ASSIGNED_CONTEXT((#170251,#170253,#170254))
REPRESENTATION_CONTEXT('','3D')
);
#170251=(
LENGTH_UNIT()
NAMED_UNIT(*)
SI_UNIT(.MILLI.,.METRE.)
);
#170253=(
NAMED_UNIT(*)
PLANE_ANGLE_UNIT()
SI_UNIT($,.RADIAN.)
);
#170254=(
NAMED_UNIT(*)
SI_UNIT($,.STERADIAN.)
SOLID_ANGLE_UNIT()
);
#170259=SHAPE_DEFINITION_REPRESENTATION(#170266,#170279);
#170266=PRODUCT_DEFINITION_SHAPE('',$,#170287);
#170279=SHAPE_REPRESENTATION('',(#77711),#170247);
#170282=PRODUCT_DEFINITION_CONTEXT('part definition',#170305,'design');
#170287=PRODUCT_DEFINITION('2026-11-14-09-55-10-334_3',
'Plunge Mounting',#170294,#170282);
#170294=PRODUCT_DEFINITION_FORMATION('',$,#170311);
#170305=APPLICATION_CONTEXT(
'Core Data for Automotive Mechanical Design Process');
#170306=PRODUCT_CONTEXT('part definition',#170305,'mechanical');
#170311=PRODUCT('2026-11-14-09-55-10-334_3','Plunge Mounting',$,(#170306));
#170315=PRESENTATION_STYLE_ASSIGNMENT((#170319));
#170319=SURFACE_STYLE_USAGE(.BOTH.,#170323);
#170323=SURFACE_SIDE_STYLE('',(#170327));
#170327=SURFACE_STYLE_FILL_AREA(#170331);
#170331=FILL_AREA_STYLE('Opaque(227,224,212)',(#170335));
#170335=FILL_AREA_STYLE_COLOUR('Opaque(227,224,212)',#170339);
#170339=COLOUR_RGB('Opaque(227,224,212)',0.890196078431372,0.87843137254902,
0.831372549019608);
ENDSEC;
END-ISO-10303-21;
